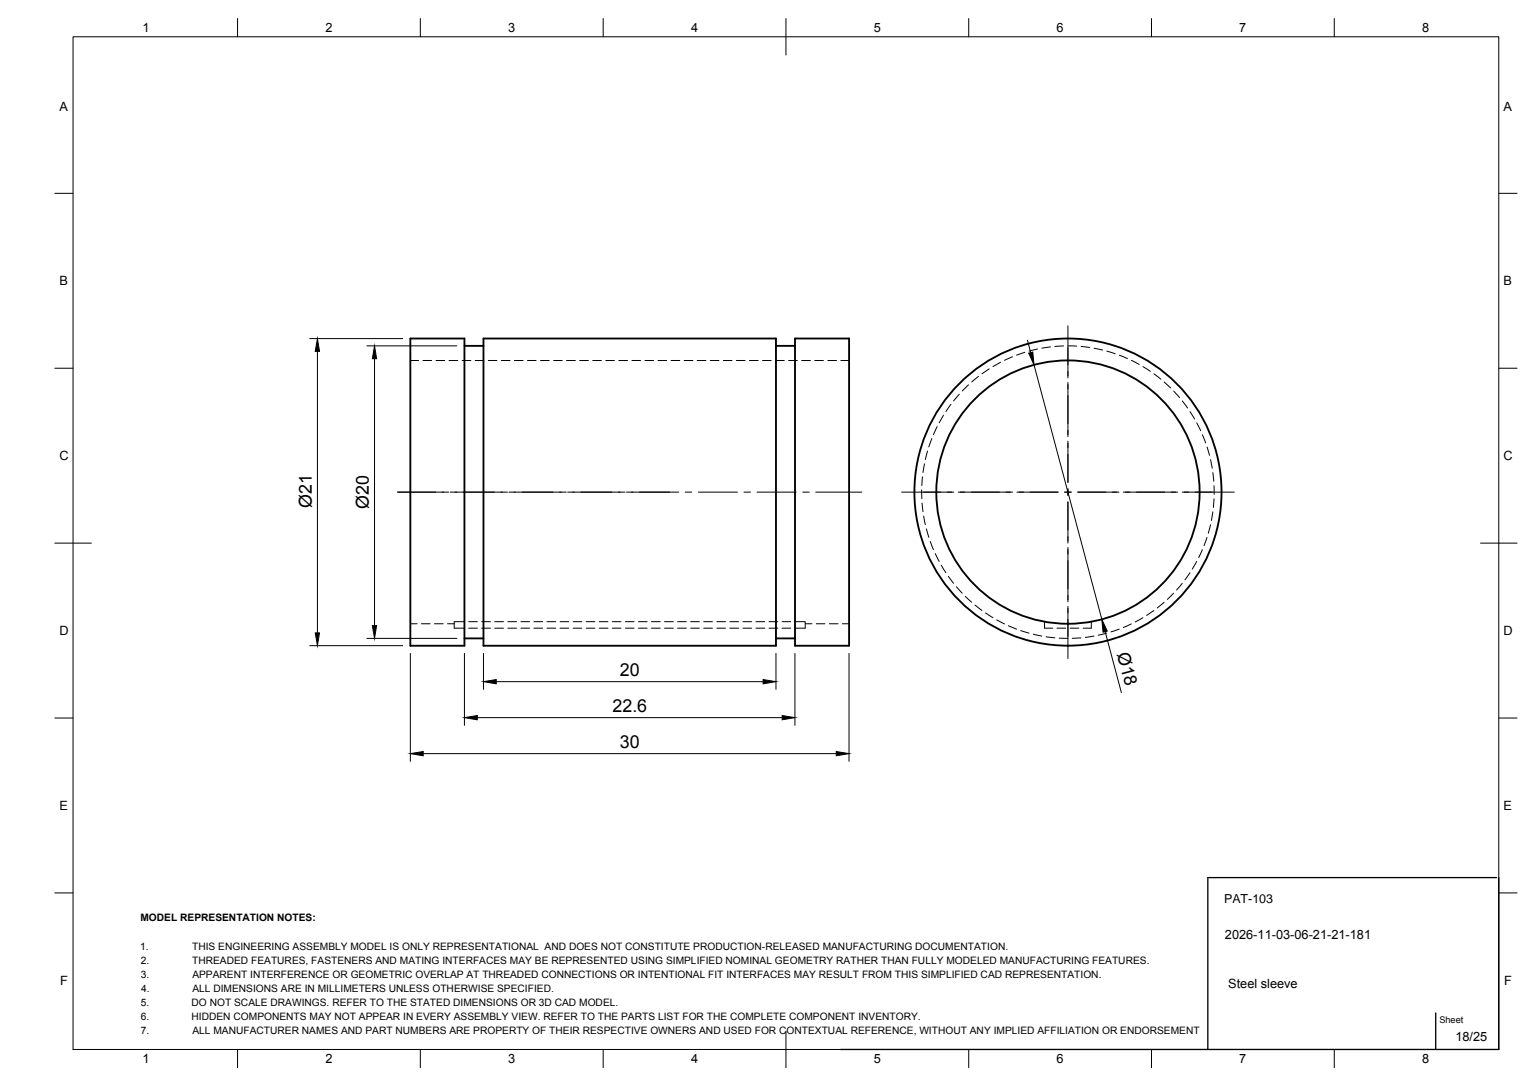
ISO-10303-21;
HEADER;
/* Generated by software containing ST-Developer
 * from STEP Tools, Inc. (www.steptools.com) 
 */

FILE_DESCRIPTION(
/* description */ ('Telescoping shaft support with lock collar'),
/* implementation_level */ '2;1');

FILE_NAME(
/* name */ 'Steel sleeve.step',
/* time_stamp */ '2026-10-27T10:48:51-07:00',
/* author */ (''),
/* organization */ (''),
/* preprocessor_version */ 'ST-DEVELOPER v20.2',
/* originating_system */ 'Autodesk Translation Framework v15.17.0.0',
/* authorisation */ '');

FILE_SCHEMA (('AUTOMOTIVE_DESIGN { 1 0 10303 214 3 1 1 }'));
ENDSEC;

DATA;
#10=MECHANICAL_DESIGN_GEOMETRIC_PRESENTATION_REPRESENTATION('',(#253),#7349);
#213=SHAPE_REPRESENTATION_RELATIONSHIP('SRR','None',#7456,#233);
#233=ADVANCED_BREP_SHAPE_REPRESENTATION('',(#272),#7340);
#253=STYLED_ITEM('',(#7641),#272);
#272=MANIFOLD_SOLID_BREP('Body1',#3977);
#338=FACE_BOUND('',#931,.T.);
#339=FACE_BOUND('',#934,.T.);
#340=FACE_BOUND('',#937,.T.);
#341=FACE_BOUND('',#940,.T.);
#342=FACE_BOUND('',#943,.T.);
#343=FACE_BOUND('',#946,.T.);
#344=FACE_BOUND('',#948,.T.);
#444=PLANE('',#4521);
#445=PLANE('',#4523);
#446=PLANE('',#4524);
#447=PLANE('',#4526);
#448=PLANE('',#4527);
#449=PLANE('',#4528);
#450=PLANE('',#4533);
#451=PLANE('',#4537);
#452=PLANE('',#4541);
#453=PLANE('',#4545);
#454=PLANE('',#4549);
#640=FACE_OUTER_BOUND('',#925,.T.);
#641=FACE_OUTER_BOUND('',#926,.T.);
#642=FACE_OUTER_BOUND('',#927,.T.);
#643=FACE_OUTER_BOUND('',#928,.T.);
#644=FACE_OUTER_BOUND('',#929,.T.);
#645=FACE_OUTER_BOUND('',#930,.T.);
#646=FACE_OUTER_BOUND('',#932,.T.);
#647=FACE_OUTER_BOUND('',#933,.T.);
#648=FACE_OUTER_BOUND('',#935,.T.);
#649=FACE_OUTER_BOUND('',#936,.T.);
#650=FACE_OUTER_BOUND('',#938,.T.);
#651=FACE_OUTER_BOUND('',#939,.T.);
#652=FACE_OUTER_BOUND('',#941,.T.);
#653=FACE_OUTER_BOUND('',#942,.T.);
#654=FACE_OUTER_BOUND('',#944,.T.);
#655=FACE_OUTER_BOUND('',#945,.T.);
#656=FACE_OUTER_BOUND('',#947,.T.);
#925=EDGE_LOOP('',(#3332,#3333,#3334,#3335));
#926=EDGE_LOOP('',(#3336,#3337,#3338,#3339));
#927=EDGE_LOOP('',(#3340,#3341,#3342,#3343));
#928=EDGE_LOOP('',(#3344,#3345,#3346,#3347));
#929=EDGE_LOOP('',(#3348,#3349,#3350,#3351));
#930=EDGE_LOOP('',(#3352));
#931=EDGE_LOOP('',(#3353));
#932=EDGE_LOOP('',(#3354,#3355,#3356,#3357));
#933=EDGE_LOOP('',(#3358));
#934=EDGE_LOOP('',(#3359));
#935=EDGE_LOOP('',(#3360,#3361,#3362,#3363));
#936=EDGE_LOOP('',(#3364));
#937=EDGE_LOOP('',(#3365));
#938=EDGE_LOOP('',(#3366,#3367,#3368,#3369));
#939=EDGE_LOOP('',(#3370));
#940=EDGE_LOOP('',(#3371));
#941=EDGE_LOOP('',(#3372,#3373,#3374,#3375));
#942=EDGE_LOOP('',(#3376));
#943=EDGE_LOOP('',(#3377));
#944=EDGE_LOOP('',(#3378,#3379,#3380,#3381));
#945=EDGE_LOOP('',(#3382));
#946=EDGE_LOOP('',(#3383));
#947=EDGE_LOOP('',(#3384,#3385,#3386,#3387));
#948=EDGE_LOOP('',(#3388,#3389,#3390,#3391));
#1215=LINE('',#6797,#1495);
#1216=LINE('',#6799,#1496);
#1217=LINE('',#6800,#1497);
#1218=LINE('',#6803,#1498);
#1219=LINE('',#6805,#1499);
#1220=LINE('',#6806,#1500);
#1221=LINE('',#6811,#1501);
#1222=LINE('',#6812,#1502);
#1223=LINE('',#6814,#1503);
#1224=LINE('',#6815,#1504);
#1225=LINE('',#6825,#1505);
#1226=LINE('',#6832,#1506);
#1227=LINE('',#6839,#1507);
#1228=LINE('',#6846,#1508);
#1229=LINE('',#6853,#1509);
#1230=LINE('',#6858,#1510);
#1495=VECTOR('',#5527,1.);
#1496=VECTOR('',#5528,1.);
#1497=VECTOR('',#5529,1.);
#1498=VECTOR('',#5532,1.);
#1499=VECTOR('',#5533,1.);
#1500=VECTOR('',#5534,1.);
#1501=VECTOR('',#5539,1.);
#1502=VECTOR('',#5540,1.);
#1503=VECTOR('',#5543,1.);
#1504=VECTOR('',#5544,1.);
#1505=VECTOR('',#5557,1.05);
#1506=VECTOR('',#5566,1.);
#1507=VECTOR('',#5575,1.05);
#1508=VECTOR('',#5584,1.);
#1509=VECTOR('',#5593,1.05);
#1510=VECTOR('',#5600,0.9);
#1740=CIRCLE('',#4522,0.9);
#1741=CIRCLE('',#4525,0.9);
#1742=CIRCLE('',#4529,1.05);
#1743=CIRCLE('',#4530,0.9);
#1744=CIRCLE('',#4532,1.05);
#1745=CIRCLE('',#4534,1.);
#1746=CIRCLE('',#4536,1.);
#1747=CIRCLE('',#4538,1.05);
#1748=CIRCLE('',#4540,1.05);
#1749=CIRCLE('',#4542,1.);
#1750=CIRCLE('',#4544,1.);
#1751=CIRCLE('',#4546,1.05);
#1752=CIRCLE('',#4548,1.05);
#1753=CIRCLE('',#4550,0.9);
#2027=VERTEX_POINT('',#6793);
#2028=VERTEX_POINT('',#6794);
#2029=VERTEX_POINT('',#6796);
#2030=VERTEX_POINT('',#6798);
#2031=VERTEX_POINT('',#6802);
#2032=VERTEX_POINT('',#6804);
#2033=VERTEX_POINT('',#6808);
#2034=VERTEX_POINT('',#6810);
#2035=VERTEX_POINT('',#6818);
#2036=VERTEX_POINT('',#6820);
#2037=VERTEX_POINT('',#6823);
#2038=VERTEX_POINT('',#6827);
#2039=VERTEX_POINT('',#6830);
#2040=VERTEX_POINT('',#6834);
#2041=VERTEX_POINT('',#6837);
#2042=VERTEX_POINT('',#6841);
#2043=VERTEX_POINT('',#6844);
#2044=VERTEX_POINT('',#6848);
#2045=VERTEX_POINT('',#6851);
#2046=VERTEX_POINT('',#6855);
#2478=EDGE_CURVE('',#2027,#2028,#1740,.T.);
#2479=EDGE_CURVE('',#2029,#2027,#1215,.T.);
#2480=EDGE_CURVE('',#2030,#2029,#1216,.T.);
#2481=EDGE_CURVE('',#2028,#2030,#1217,.T.);
#2482=EDGE_CURVE('',#2028,#2031,#1218,.T.);
#2483=EDGE_CURVE('',#2032,#2030,#1219,.T.);
#2484=EDGE_CURVE('',#2032,#2031,#1220,.T.);
#2485=EDGE_CURVE('',#2031,#2033,#1741,.T.);
#2486=EDGE_CURVE('',#2034,#2032,#1221,.T.);
#2487=EDGE_CURVE('',#2033,#2034,#1222,.T.);
#2488=EDGE_CURVE('',#2033,#2027,#1223,.T.);
#2489=EDGE_CURVE('',#2034,#2029,#1224,.T.);
#2490=EDGE_CURVE('',#2035,#2035,#1742,.T.);
#2491=EDGE_CURVE('',#2036,#2036,#1743,.T.);
#2492=EDGE_CURVE('',#2037,#2037,#1744,.T.);
#2493=EDGE_CURVE('',#2037,#2035,#1225,.T.);
#2494=EDGE_CURVE('',#2038,#2038,#1745,.T.);
#2495=EDGE_CURVE('',#2039,#2039,#1746,.T.);
#2496=EDGE_CURVE('',#2039,#2038,#1226,.T.);
#2497=EDGE_CURVE('',#2040,#2040,#1747,.T.);
#2498=EDGE_CURVE('',#2041,#2041,#1748,.T.);
#2499=EDGE_CURVE('',#2041,#2040,#1227,.T.);
#2500=EDGE_CURVE('',#2042,#2042,#1749,.T.);
#2501=EDGE_CURVE('',#2043,#2043,#1750,.T.);
#2502=EDGE_CURVE('',#2043,#2042,#1228,.T.);
#2503=EDGE_CURVE('',#2044,#2044,#1751,.T.);
#2504=EDGE_CURVE('',#2045,#2045,#1752,.T.);
#2505=EDGE_CURVE('',#2045,#2044,#1229,.T.);
#2506=EDGE_CURVE('',#2046,#2046,#1753,.T.);
#2507=EDGE_CURVE('',#2046,#2036,#1230,.T.);
#3332=ORIENTED_EDGE('',*,*,#2478,.F.);
#3333=ORIENTED_EDGE('',*,*,#2479,.F.);
#3334=ORIENTED_EDGE('',*,*,#2480,.F.);
#3335=ORIENTED_EDGE('',*,*,#2481,.F.);
#3336=ORIENTED_EDGE('',*,*,#2482,.F.);
#3337=ORIENTED_EDGE('',*,*,#2481,.T.);
#3338=ORIENTED_EDGE('',*,*,#2483,.F.);
#3339=ORIENTED_EDGE('',*,*,#2484,.T.);
#3340=ORIENTED_EDGE('',*,*,#2485,.F.);
#3341=ORIENTED_EDGE('',*,*,#2484,.F.);
#3342=ORIENTED_EDGE('',*,*,#2486,.F.);
#3343=ORIENTED_EDGE('',*,*,#2487,.F.);
#3344=ORIENTED_EDGE('',*,*,#2488,.F.);
#3345=ORIENTED_EDGE('',*,*,#2487,.T.);
#3346=ORIENTED_EDGE('',*,*,#2489,.T.);
#3347=ORIENTED_EDGE('',*,*,#2479,.T.);
#3348=ORIENTED_EDGE('',*,*,#2489,.F.);
#3349=ORIENTED_EDGE('',*,*,#2486,.T.);
#3350=ORIENTED_EDGE('',*,*,#2483,.T.);
#3351=ORIENTED_EDGE('',*,*,#2480,.T.);
#3352=ORIENTED_EDGE('',*,*,#2490,.F.);
#3353=ORIENTED_EDGE('',*,*,#2491,.T.);
#3354=ORIENTED_EDGE('',*,*,#2492,.F.);
#3355=ORIENTED_EDGE('',*,*,#2493,.T.);
#3356=ORIENTED_EDGE('',*,*,#2490,.T.);
#3357=ORIENTED_EDGE('',*,*,#2493,.F.);
#3358=ORIENTED_EDGE('',*,*,#2492,.T.);
#3359=ORIENTED_EDGE('',*,*,#2494,.F.);
#3360=ORIENTED_EDGE('',*,*,#2495,.F.);
#3361=ORIENTED_EDGE('',*,*,#2496,.T.);
#3362=ORIENTED_EDGE('',*,*,#2494,.T.);
#3363=ORIENTED_EDGE('',*,*,#2496,.F.);
#3364=ORIENTED_EDGE('',*,*,#2497,.F.);
#3365=ORIENTED_EDGE('',*,*,#2495,.T.);
#3366=ORIENTED_EDGE('',*,*,#2498,.F.);
#3367=ORIENTED_EDGE('',*,*,#2499,.T.);
#3368=ORIENTED_EDGE('',*,*,#2497,.T.);
#3369=ORIENTED_EDGE('',*,*,#2499,.F.);
#3370=ORIENTED_EDGE('',*,*,#2498,.T.);
#3371=ORIENTED_EDGE('',*,*,#2500,.F.);
#3372=ORIENTED_EDGE('',*,*,#2501,.F.);
#3373=ORIENTED_EDGE('',*,*,#2502,.T.);
#3374=ORIENTED_EDGE('',*,*,#2500,.T.);
#3375=ORIENTED_EDGE('',*,*,#2502,.F.);
#3376=ORIENTED_EDGE('',*,*,#2503,.F.);
#3377=ORIENTED_EDGE('',*,*,#2501,.T.);
#3378=ORIENTED_EDGE('',*,*,#2504,.F.);
#3379=ORIENTED_EDGE('',*,*,#2505,.T.);
#3380=ORIENTED_EDGE('',*,*,#2503,.T.);
#3381=ORIENTED_EDGE('',*,*,#2505,.F.);
#3382=ORIENTED_EDGE('',*,*,#2504,.T.);
#3383=ORIENTED_EDGE('',*,*,#2506,.F.);
#3384=ORIENTED_EDGE('',*,*,#2506,.T.);
#3385=ORIENTED_EDGE('',*,*,#2507,.T.);
#3386=ORIENTED_EDGE('',*,*,#2491,.F.);
#3387=ORIENTED_EDGE('',*,*,#2507,.F.);
#3388=ORIENTED_EDGE('',*,*,#2485,.T.);
#3389=ORIENTED_EDGE('',*,*,#2488,.T.);
#3390=ORIENTED_EDGE('',*,*,#2478,.T.);
#3391=ORIENTED_EDGE('',*,*,#2482,.T.);
#3716=CYLINDRICAL_SURFACE('',#4531,1.05);
#3717=CYLINDRICAL_SURFACE('',#4535,1.);
#3718=CYLINDRICAL_SURFACE('',#4539,1.05);
#3719=CYLINDRICAL_SURFACE('',#4543,1.);
#3720=CYLINDRICAL_SURFACE('',#4547,1.05);
#3721=CYLINDRICAL_SURFACE('',#4551,0.9);
#3883=ADVANCED_FACE('',(#640),#444,.F.);
#3884=ADVANCED_FACE('',(#641),#445,.F.);
#3885=ADVANCED_FACE('',(#642),#446,.F.);
#3886=ADVANCED_FACE('',(#643),#447,.F.);
#3887=ADVANCED_FACE('',(#644),#448,.F.);
#3888=ADVANCED_FACE('',(#645,#338),#449,.T.);
#3889=ADVANCED_FACE('',(#646),#3716,.T.);
#3890=ADVANCED_FACE('',(#647,#339),#450,.T.);
#3891=ADVANCED_FACE('',(#648),#3717,.T.);
#3892=ADVANCED_FACE('',(#649,#340),#451,.T.);
#3893=ADVANCED_FACE('',(#650),#3718,.T.);
#3894=ADVANCED_FACE('',(#651,#341),#452,.T.);
#3895=ADVANCED_FACE('',(#652),#3719,.T.);
#3896=ADVANCED_FACE('',(#653,#342),#453,.T.);
#3897=ADVANCED_FACE('',(#654),#3720,.T.);
#3898=ADVANCED_FACE('',(#655,#343),#454,.T.);
#3899=ADVANCED_FACE('',(#656,#344),#3721,.F.);
#3977=CLOSED_SHELL('',(#3883,#3884,#3885,#3886,#3887,#3888,#3889,#3890,
#3891,#3892,#3893,#3894,#3895,#3896,#3897,#3898,#3899));
#4520=AXIS2_PLACEMENT_3D('',#6791,#5521,#5522);
#4521=AXIS2_PLACEMENT_3D('',#6792,#5523,#5524);
#4522=AXIS2_PLACEMENT_3D('',#6795,#5525,#5526);
#4523=AXIS2_PLACEMENT_3D('',#6801,#5530,#5531);
#4524=AXIS2_PLACEMENT_3D('',#6807,#5535,#5536);
#4525=AXIS2_PLACEMENT_3D('',#6809,#5537,#5538);
#4526=AXIS2_PLACEMENT_3D('',#6813,#5541,#5542);
#4527=AXIS2_PLACEMENT_3D('',#6816,#5545,#5546);
#4528=AXIS2_PLACEMENT_3D('',#6817,#5547,#5548);
#4529=AXIS2_PLACEMENT_3D('',#6819,#5549,#5550);
#4530=AXIS2_PLACEMENT_3D('',#6821,#5551,#5552);
#4531=AXIS2_PLACEMENT_3D('',#6822,#5553,#5554);
#4532=AXIS2_PLACEMENT_3D('',#6824,#5555,#5556);
#4533=AXIS2_PLACEMENT_3D('',#6826,#5558,#5559);
#4534=AXIS2_PLACEMENT_3D('',#6828,#5560,#5561);
#4535=AXIS2_PLACEMENT_3D('',#6829,#5562,#5563);
#4536=AXIS2_PLACEMENT_3D('',#6831,#5564,#5565);
#4537=AXIS2_PLACEMENT_3D('',#6833,#5567,#5568);
#4538=AXIS2_PLACEMENT_3D('',#6835,#5569,#5570);
#4539=AXIS2_PLACEMENT_3D('',#6836,#5571,#5572);
#4540=AXIS2_PLACEMENT_3D('',#6838,#5573,#5574);
#4541=AXIS2_PLACEMENT_3D('',#6840,#5576,#5577);
#4542=AXIS2_PLACEMENT_3D('',#6842,#5578,#5579);
#4543=AXIS2_PLACEMENT_3D('',#6843,#5580,#5581);
#4544=AXIS2_PLACEMENT_3D('',#6845,#5582,#5583);
#4545=AXIS2_PLACEMENT_3D('',#6847,#5585,#5586);
#4546=AXIS2_PLACEMENT_3D('',#6849,#5587,#5588);
#4547=AXIS2_PLACEMENT_3D('',#6850,#5589,#5590);
#4548=AXIS2_PLACEMENT_3D('',#6852,#5591,#5592);
#4549=AXIS2_PLACEMENT_3D('',#6854,#5594,#5595);
#4550=AXIS2_PLACEMENT_3D('',#6856,#5596,#5597);
#4551=AXIS2_PLACEMENT_3D('',#6857,#5598,#5599);
#5521=DIRECTION('axis',(0.,0.,1.));
#5522=DIRECTION('refdir',(1.,0.,0.));
#5523=DIRECTION('center_axis',(0.,1.,0.));
#5524=DIRECTION('ref_axis',(0.,0.,1.));
#5525=DIRECTION('center_axis',(0.,-1.,0.));
#5526=DIRECTION('ref_axis',(1.,0.,0.));
#5527=DIRECTION('',(-1.,0.,0.));
#5528=DIRECTION('',(0.,0.,-1.));
#5529=DIRECTION('',(1.,0.,0.));
#5530=DIRECTION('center_axis',(0.,0.,1.));
#5531=DIRECTION('ref_axis',(1.,0.,0.));
#5532=DIRECTION('',(0.,-1.,0.));
#5533=DIRECTION('',(0.,1.,0.));
#5534=DIRECTION('',(-1.,0.,0.));
#5535=DIRECTION('center_axis',(0.,-1.,0.));
#5536=DIRECTION('ref_axis',(0.,0.,-1.));
#5537=DIRECTION('center_axis',(0.,1.,0.));
#5538=DIRECTION('ref_axis',(1.,0.,0.));
#5539=DIRECTION('',(0.,0.,1.));
#5540=DIRECTION('',(1.,0.,0.));
#5541=DIRECTION('center_axis',(0.,0.,-1.));
#5542=DIRECTION('ref_axis',(-1.,0.,0.));
#5543=DIRECTION('',(0.,1.,0.));
#5544=DIRECTION('',(0.,1.,0.));
#5545=DIRECTION('center_axis',(1.,0.,0.));
#5546=DIRECTION('ref_axis',(0.,0.,-1.));
#5547=DIRECTION('center_axis',(0.,1.,0.));
#5548=DIRECTION('ref_axis',(0.,0.,1.));
#5549=DIRECTION('center_axis',(0.,-1.,0.));
#5550=DIRECTION('ref_axis',(1.,0.,0.));
#5551=DIRECTION('center_axis',(0.,-1.,0.));
#5552=DIRECTION('ref_axis',(1.,0.,0.));
#5553=DIRECTION('center_axis',(0.,-1.,0.));
#5554=DIRECTION('ref_axis',(1.,0.,0.));
#5555=DIRECTION('center_axis',(0.,-1.,0.));
#5556=DIRECTION('ref_axis',(1.,0.,0.));
#5557=DIRECTION('',(0.,1.,0.));
#5558=DIRECTION('center_axis',(0.,-1.,0.));
#5559=DIRECTION('ref_axis',(0.,0.,-1.));
#5560=DIRECTION('center_axis',(0.,-1.,0.));
#5561=DIRECTION('ref_axis',(1.,0.,0.));
#5562=DIRECTION('center_axis',(0.,-1.,0.));
#5563=DIRECTION('ref_axis',(1.,0.,0.));
#5564=DIRECTION('center_axis',(0.,-1.,0.));
#5565=DIRECTION('ref_axis',(1.,0.,0.));
#5566=DIRECTION('',(0.,1.,0.));
#5567=DIRECTION('center_axis',(0.,1.,0.));
#5568=DIRECTION('ref_axis',(0.,0.,1.));
#5569=DIRECTION('center_axis',(0.,-1.,0.));
#5570=DIRECTION('ref_axis',(1.,0.,0.));
#5571=DIRECTION('center_axis',(0.,-1.,0.));
#5572=DIRECTION('ref_axis',(1.,0.,0.));
#5573=DIRECTION('center_axis',(0.,-1.,0.));
#5574=DIRECTION('ref_axis',(1.,0.,0.));
#5575=DIRECTION('',(0.,1.,0.));
#5576=DIRECTION('center_axis',(0.,-1.,0.));
#5577=DIRECTION('ref_axis',(0.,0.,-1.));
#5578=DIRECTION('center_axis',(0.,-1.,0.));
#5579=DIRECTION('ref_axis',(1.,0.,0.));
#5580=DIRECTION('center_axis',(0.,-1.,0.));
#5581=DIRECTION('ref_axis',(1.,0.,0.));
#5582=DIRECTION('center_axis',(0.,-1.,0.));
#5583=DIRECTION('ref_axis',(1.,0.,0.));
#5584=DIRECTION('',(0.,1.,0.));
#5585=DIRECTION('center_axis',(0.,1.,0.));
#5586=DIRECTION('ref_axis',(0.,0.,1.));
#5587=DIRECTION('center_axis',(0.,-1.,0.));
#5588=DIRECTION('ref_axis',(1.,0.,0.));
#5589=DIRECTION('center_axis',(0.,-1.,0.));
#5590=DIRECTION('ref_axis',(1.,0.,0.));
#5591=DIRECTION('center_axis',(0.,-1.,0.));
#5592=DIRECTION('ref_axis',(1.,0.,0.));
#5593=DIRECTION('',(0.,1.,0.));
#5594=DIRECTION('center_axis',(0.,-1.,0.));
#5595=DIRECTION('ref_axis',(0.,0.,-1.));
#5596=DIRECTION('center_axis',(0.,-1.,0.));
#5597=DIRECTION('ref_axis',(1.,0.,0.));
#5598=DIRECTION('center_axis',(0.,-1.,0.));
#5599=DIRECTION('ref_axis',(1.,0.,0.));
#5600=DIRECTION('',(0.,1.,0.));
#6791=CARTESIAN_POINT('',(0.,0.,0.));
#6792=CARTESIAN_POINT('Origin',(0.75,1.2,0.));
#6793=CARTESIAN_POINT('',(0.885663593019381,1.2,-0.16));
#6794=CARTESIAN_POINT('',(0.885663593019381,1.2,0.16));
#6795=CARTESIAN_POINT('Origin',(0.,1.2,0.));
#6796=CARTESIAN_POINT('',(0.93,1.2,-0.16));
#6797=CARTESIAN_POINT('',(0.93,1.2,-0.16));
#6798=CARTESIAN_POINT('',(0.93,1.2,0.16));
#6799=CARTESIAN_POINT('',(0.93,1.2,0.16));
#6800=CARTESIAN_POINT('',(0.57,1.2,0.16));
#6801=CARTESIAN_POINT('Origin',(0.57,0.,0.16));
#6802=CARTESIAN_POINT('',(0.885663593019381,-1.2,0.16));
#6803=CARTESIAN_POINT('',(0.885663593019381,0.,0.16));
#6804=CARTESIAN_POINT('',(0.93,-1.2,0.16));
#6805=CARTESIAN_POINT('',(0.93,0.,0.16));
#6806=CARTESIAN_POINT('',(0.57,-1.2,0.16));
#6807=CARTESIAN_POINT('Origin',(0.75,-1.2,0.));
#6808=CARTESIAN_POINT('',(0.885663593019381,-1.2,-0.16));
#6809=CARTESIAN_POINT('Origin',(0.,-1.2,0.));
#6810=CARTESIAN_POINT('',(0.93,-1.2,-0.16));
#6811=CARTESIAN_POINT('',(0.93,-1.2,0.16));
#6812=CARTESIAN_POINT('',(0.93,-1.2,-0.16));
#6813=CARTESIAN_POINT('Origin',(0.93,0.,-0.16));
#6814=CARTESIAN_POINT('',(0.885663593019381,0.,-0.16));
#6815=CARTESIAN_POINT('',(0.93,0.,-0.16));
#6816=CARTESIAN_POINT('Origin',(0.93,0.,0.16));
#6817=CARTESIAN_POINT('Origin',(1.05,1.5,0.));
#6818=CARTESIAN_POINT('',(-1.05,1.5,-1.28587913910472E-16));
#6819=CARTESIAN_POINT('Origin',(0.,1.5,0.));
#6820=CARTESIAN_POINT('',(-0.9,1.5,-1.10218211923262E-16));
#6821=CARTESIAN_POINT('Origin',(0.,1.5,0.));
#6822=CARTESIAN_POINT('Origin',(0.,1.315,0.));
#6823=CARTESIAN_POINT('',(-1.05,1.13,-1.28587913910472E-16));
#6824=CARTESIAN_POINT('Origin',(0.,1.13,0.));
#6825=CARTESIAN_POINT('',(-1.05,1.315,-1.28587913910472E-16));
#6826=CARTESIAN_POINT('Origin',(1.,1.13,0.));
#6827=CARTESIAN_POINT('',(-1.,1.13,-1.22464679914735E-16));
#6828=CARTESIAN_POINT('Origin',(0.,1.13,0.));
#6829=CARTESIAN_POINT('Origin',(0.,1.065,0.));
#6830=CARTESIAN_POINT('',(-1.,1.,-1.22464679914735E-16));
#6831=CARTESIAN_POINT('Origin',(0.,1.,0.));
#6832=CARTESIAN_POINT('',(-1.,1.065,-1.22464679914735E-16));
#6833=CARTESIAN_POINT('Origin',(1.05,1.,0.));
#6834=CARTESIAN_POINT('',(-1.05,1.,-1.28587913910472E-16));
#6835=CARTESIAN_POINT('Origin',(0.,1.,0.));
#6836=CARTESIAN_POINT('Origin',(0.,0.,0.));
#6837=CARTESIAN_POINT('',(-1.05,-1.,-1.28587913910472E-16));
#6838=CARTESIAN_POINT('Origin',(0.,-1.,0.));
#6839=CARTESIAN_POINT('',(-1.05,0.,-1.28587913910472E-16));
#6840=CARTESIAN_POINT('Origin',(1.,-1.,0.));
#6841=CARTESIAN_POINT('',(-1.,-1.,-1.22464679914735E-16));
#6842=CARTESIAN_POINT('Origin',(0.,-1.,0.));
#6843=CARTESIAN_POINT('Origin',(0.,-1.065,0.));
#6844=CARTESIAN_POINT('',(-1.,-1.13,-1.22464679914735E-16));
#6845=CARTESIAN_POINT('Origin',(0.,-1.13,0.));
#6846=CARTESIAN_POINT('',(-1.,-1.065,-1.22464679914735E-16));
#6847=CARTESIAN_POINT('Origin',(1.05,-1.13,0.));
#6848=CARTESIAN_POINT('',(-1.05,-1.13,-1.28587913910472E-16));
#6849=CARTESIAN_POINT('Origin',(0.,-1.13,0.));
#6850=CARTESIAN_POINT('Origin',(0.,-1.315,0.));
#6851=CARTESIAN_POINT('',(-1.05,-1.5,-1.28587913910472E-16));
#6852=CARTESIAN_POINT('Origin',(0.,-1.5,0.));
#6853=CARTESIAN_POINT('',(-1.05,-1.315,-1.28587913910472E-16));
#6854=CARTESIAN_POINT('Origin',(0.9,-1.5,0.));
#6855=CARTESIAN_POINT('',(-0.9,-1.5,-1.10218211923262E-16));
#6856=CARTESIAN_POINT('Origin',(0.,-1.5,0.));
#6857=CARTESIAN_POINT('Origin',(0.,0.,0.));
#6858=CARTESIAN_POINT('',(-0.9,0.,-1.10218211923262E-16));
#7315=UNCERTAINTY_MEASURE_WITH_UNIT(LENGTH_MEASURE(0.001),#7350,
'DISTANCE_ACCURACY_VALUE',
'Maximum model space distance between geometric entities at asserted c
onnectivities');
#7324=UNCERTAINTY_MEASURE_WITH_UNIT(LENGTH_MEASURE(0.001),#7350,
'DISTANCE_ACCURACY_VALUE',
'Maximum model space distance between geometric entities at asserted c
onnectivities');
#7340=(
GEOMETRIC_REPRESENTATION_CONTEXT(3)
GLOBAL_UNCERTAINTY_ASSIGNED_CONTEXT((#7315))
GLOBAL_UNIT_ASSIGNED_CONTEXT((#7350,#7352,#7353))
REPRESENTATION_CONTEXT('','3D')
);
#7349=(
GEOMETRIC_REPRESENTATION_CONTEXT(3)
GLOBAL_UNCERTAINTY_ASSIGNED_CONTEXT((#7324))
GLOBAL_UNIT_ASSIGNED_CONTEXT((#7350,#7352,#7353))
REPRESENTATION_CONTEXT('','3D')
);
#7350=(
LENGTH_UNIT()
NAMED_UNIT(*)
SI_UNIT(.CENTI.,.METRE.)
);
#7352=(
NAMED_UNIT(*)
PLANE_ANGLE_UNIT()
SI_UNIT($,.RADIAN.)
);
#7353=(
NAMED_UNIT(*)
SI_UNIT($,.STERADIAN.)
SOLID_ANGLE_UNIT()
);
#7369=SHAPE_DEFINITION_REPRESENTATION(#7393,#7456);
#7393=PRODUCT_DEFINITION_SHAPE('',$,#7481);
#7456=SHAPE_REPRESENTATION('',(#4520),#7340);
#7465=PRODUCT_DEFINITION_CONTEXT('part definition',#7539,'design');
#7481=PRODUCT_DEFINITION('Steel sleeve','Steel sleeve',#7505,#7465);
#7505=PRODUCT_DEFINITION_FORMATION('',$,#7556);
#7539=APPLICATION_CONTEXT(
'Core Data for Automotive Mechanical Design Process');
#7540=PRODUCT_CONTEXT('part definition',#7539,'mechanical');
#7556=PRODUCT('Steel sleeve','Steel sleeve','Steel sleeve',(#7540));
#7635=COLOUR_RGB('Off White',0.89,0.88,0.83);
#7636=FILL_AREA_STYLE_COLOUR('',#7635);
#7637=FILL_AREA_STYLE('',(#7636));
#7638=SURFACE_STYLE_FILL_AREA(#7637);
#7639=SURFACE_SIDE_STYLE('',(#7638));
#7640=SURFACE_STYLE_USAGE(.BOTH.,#7639);
#7641=PRESENTATION_STYLE_ASSIGNMENT((#7640));
ENDSEC;
END-ISO-10303-21;
